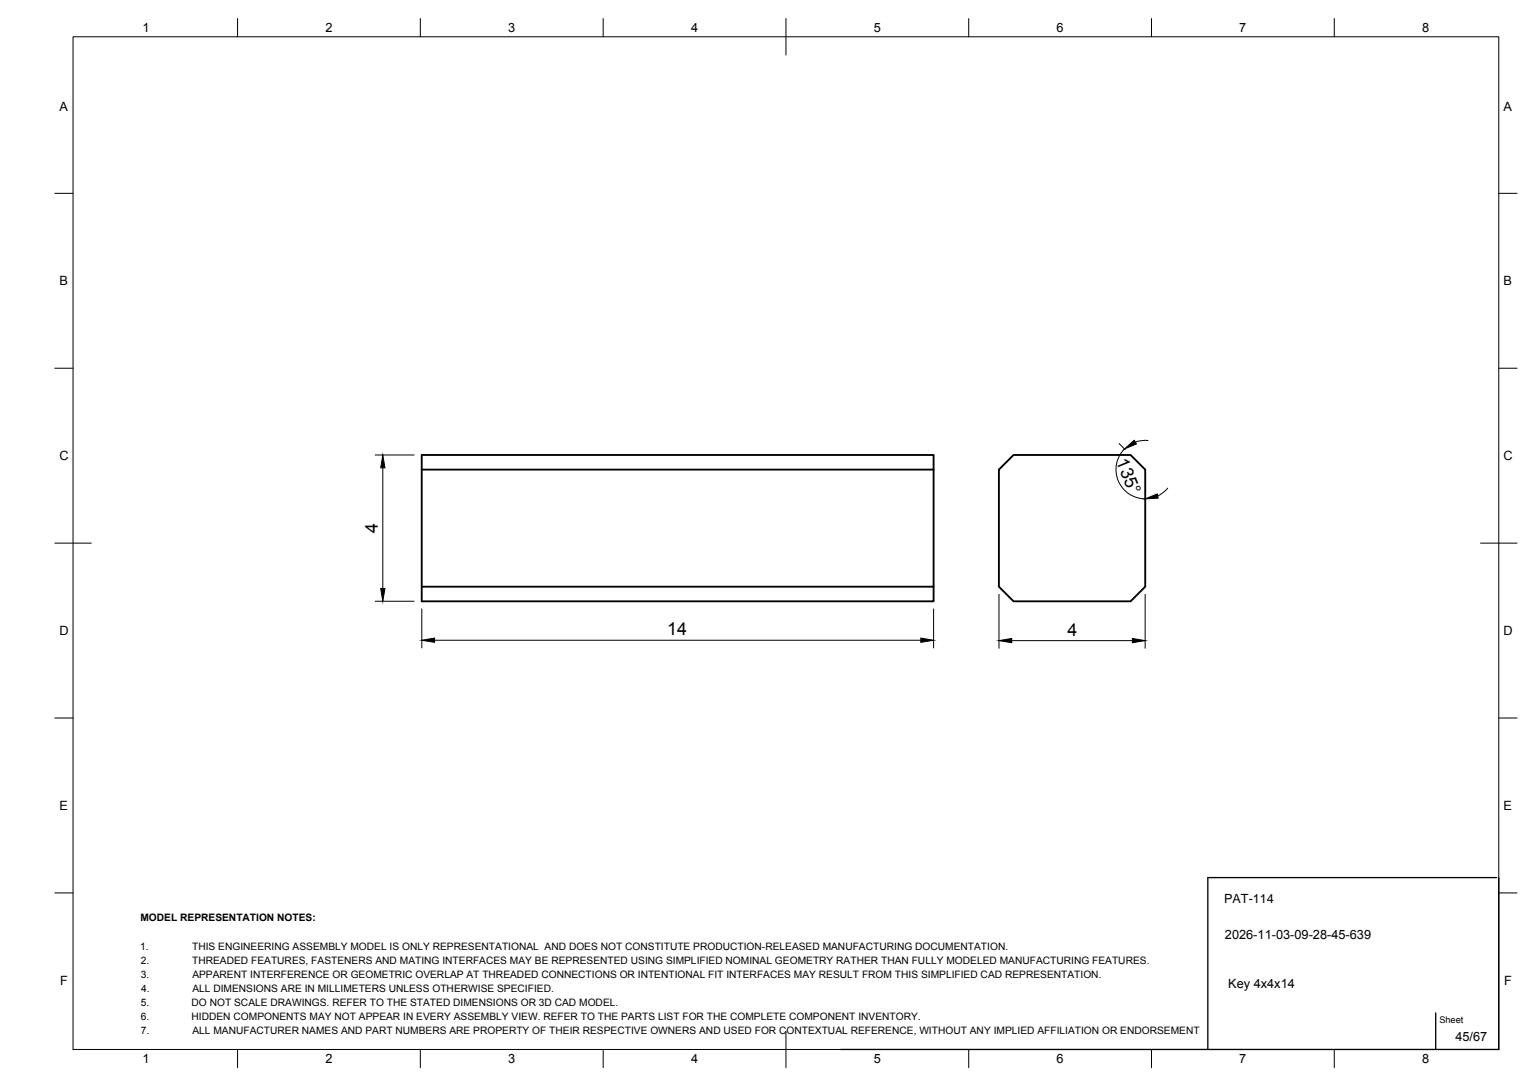
ISO-10303-21;
HEADER;
/* Generated by software containing ST-Developer
 * from STEP Tools, Inc. (www.steptools.com) 
 */

FILE_DESCRIPTION(
/* description */ ('Two-stage gear reducer in split housing'),
/* implementation_level */ '2;1');

FILE_NAME(
/* name */ 'Key 4x4x14.step',
/* time_stamp */ '2026-10-28T03:22:31-07:00',
/* author */ (''),
/* organization */ (''),
/* preprocessor_version */ 'ST-DEVELOPER v20.2',
/* originating_system */ 'Autodesk Translation Framework v15.17.0.0',
/* authorisation */ '');

FILE_SCHEMA (('AUTOMOTIVE_DESIGN { 1 0 10303 214 3 1 1 }'));
ENDSEC;

DATA;
#10=MECHANICAL_DESIGN_GEOMETRIC_PRESENTATION_REPRESENTATION('',(#1285),#73366);
#1158=SHAPE_REPRESENTATION_RELATIONSHIP('SRR','None',#73648,#1214);
#1214=ADVANCED_BREP_SHAPE_REPRESENTATION('',(#1354),#73344);
#1285=STYLED_ITEM('',(#73988),#1354);
#1354=MANIFOLD_SOLID_BREP('Body1',#16175);
#1848=PLANE('',#17938);
#1849=PLANE('',#17939);
#1850=PLANE('',#17940);
#1851=PLANE('',#17941);
#1852=PLANE('',#17942);
#1853=PLANE('',#17943);
#1854=PLANE('',#17944);
#1855=PLANE('',#17945);
#1856=PLANE('',#17946);
#1857=PLANE('',#17947);
#2542=FACE_OUTER_BOUND('',#3639,.T.);
#2543=FACE_OUTER_BOUND('',#3640,.T.);
#2544=FACE_OUTER_BOUND('',#3641,.T.);
#2545=FACE_OUTER_BOUND('',#3642,.T.);
#2546=FACE_OUTER_BOUND('',#3643,.T.);
#2547=FACE_OUTER_BOUND('',#3644,.T.);
#2548=FACE_OUTER_BOUND('',#3645,.T.);
#2549=FACE_OUTER_BOUND('',#3646,.T.);
#2550=FACE_OUTER_BOUND('',#3647,.T.);
#2551=FACE_OUTER_BOUND('',#3648,.T.);
#3639=EDGE_LOOP('',(#12941,#12942,#12943,#12944,#12945,#12946,#12947,#12948));
#3640=EDGE_LOOP('',(#12949,#12950,#12951,#12952));
#3641=EDGE_LOOP('',(#12953,#12954,#12955,#12956));
#3642=EDGE_LOOP('',(#12957,#12958,#12959,#12960));
#3643=EDGE_LOOP('',(#12961,#12962,#12963,#12964));
#3644=EDGE_LOOP('',(#12965,#12966,#12967,#12968,#12969,#12970,#12971,#12972));
#3645=EDGE_LOOP('',(#12973,#12974,#12975,#12976));
#3646=EDGE_LOOP('',(#12977,#12978,#12979,#12980));
#3647=EDGE_LOOP('',(#12981,#12982,#12983,#12984));
#3648=EDGE_LOOP('',(#12985,#12986,#12987,#12988));
#4639=LINE('',#37289,#5663);
#4640=LINE('',#37291,#5664);
#4641=LINE('',#37293,#5665);
#4642=LINE('',#37295,#5666);
#4643=LINE('',#37297,#5667);
#4644=LINE('',#37299,#5668);
#4645=LINE('',#37301,#5669);
#4646=LINE('',#37302,#5670);
#4647=LINE('',#37305,#5671);
#4648=LINE('',#37307,#5672);
#4649=LINE('',#37308,#5673);
#4650=LINE('',#37311,#5674);
#4651=LINE('',#37312,#5675);
#4652=LINE('',#37315,#5676);
#4653=LINE('',#37316,#5677);
#4654=LINE('',#37319,#5678);
#4655=LINE('',#37320,#5679);
#4656=LINE('',#37323,#5680);
#4657=LINE('',#37325,#5681);
#4658=LINE('',#37327,#5682);
#4659=LINE('',#37328,#5683);
#4660=LINE('',#37330,#5684);
#4661=LINE('',#37332,#5685);
#4662=LINE('',#37334,#5686);
#5663=VECTOR('',#21295,1.);
#5664=VECTOR('',#21296,1.);
#5665=VECTOR('',#21297,1.);
#5666=VECTOR('',#21298,1.);
#5667=VECTOR('',#21299,1.);
#5668=VECTOR('',#21300,1.);
#5669=VECTOR('',#21301,1.);
#5670=VECTOR('',#21302,1.);
#5671=VECTOR('',#21305,1.);
#5672=VECTOR('',#21306,1.);
#5673=VECTOR('',#21307,1.);
#5674=VECTOR('',#21310,1.);
#5675=VECTOR('',#21311,1.);
#5676=VECTOR('',#21314,1.);
#5677=VECTOR('',#21315,1.);
#5678=VECTOR('',#21318,1.);
#5679=VECTOR('',#21319,1.);
#5680=VECTOR('',#21322,1.);
#5681=VECTOR('',#21323,1.);
#5682=VECTOR('',#21324,1.);
#5683=VECTOR('',#21325,1.);
#5684=VECTOR('',#21328,1.);
#5685=VECTOR('',#21331,1.);
#5686=VECTOR('',#21334,1.);
#7651=VERTEX_POINT('',#37287);
#7652=VERTEX_POINT('',#37288);
#7653=VERTEX_POINT('',#37290);
#7654=VERTEX_POINT('',#37292);
#7655=VERTEX_POINT('',#37294);
#7656=VERTEX_POINT('',#37296);
#7657=VERTEX_POINT('',#37298);
#7658=VERTEX_POINT('',#37300);
#7659=VERTEX_POINT('',#37304);
#7660=VERTEX_POINT('',#37306);
#7661=VERTEX_POINT('',#37310);
#7662=VERTEX_POINT('',#37314);
#7663=VERTEX_POINT('',#37318);
#7664=VERTEX_POINT('',#37322);
#7665=VERTEX_POINT('',#37324);
#7666=VERTEX_POINT('',#37326);
#9524=EDGE_CURVE('',#7651,#7652,#4639,.T.);
#9525=EDGE_CURVE('',#7653,#7651,#4640,.T.);
#9526=EDGE_CURVE('',#7654,#7653,#4641,.T.);
#9527=EDGE_CURVE('',#7655,#7654,#4642,.T.);
#9528=EDGE_CURVE('',#7656,#7655,#4643,.T.);
#9529=EDGE_CURVE('',#7657,#7656,#4644,.T.);
#9530=EDGE_CURVE('',#7658,#7657,#4645,.T.);
#9531=EDGE_CURVE('',#7652,#7658,#4646,.T.);
#9532=EDGE_CURVE('',#7655,#7659,#4647,.T.);
#9533=EDGE_CURVE('',#7659,#7660,#4648,.T.);
#9534=EDGE_CURVE('',#7660,#7656,#4649,.T.);
#9535=EDGE_CURVE('',#7661,#7654,#4650,.T.);
#9536=EDGE_CURVE('',#7661,#7659,#4651,.T.);
#9537=EDGE_CURVE('',#7653,#7662,#4652,.T.);
#9538=EDGE_CURVE('',#7662,#7661,#4653,.T.);
#9539=EDGE_CURVE('',#7663,#7651,#4654,.T.);
#9540=EDGE_CURVE('',#7663,#7662,#4655,.T.);
#9541=EDGE_CURVE('',#7664,#7663,#4656,.T.);
#9542=EDGE_CURVE('',#7665,#7664,#4657,.T.);
#9543=EDGE_CURVE('',#7666,#7665,#4658,.T.);
#9544=EDGE_CURVE('',#7660,#7666,#4659,.T.);
#9545=EDGE_CURVE('',#7652,#7664,#4660,.T.);
#9546=EDGE_CURVE('',#7665,#7658,#4661,.T.);
#9547=EDGE_CURVE('',#7657,#7666,#4662,.T.);
#12941=ORIENTED_EDGE('',*,*,#9524,.F.);
#12942=ORIENTED_EDGE('',*,*,#9525,.F.);
#12943=ORIENTED_EDGE('',*,*,#9526,.F.);
#12944=ORIENTED_EDGE('',*,*,#9527,.F.);
#12945=ORIENTED_EDGE('',*,*,#9528,.F.);
#12946=ORIENTED_EDGE('',*,*,#9529,.F.);
#12947=ORIENTED_EDGE('',*,*,#9530,.F.);
#12948=ORIENTED_EDGE('',*,*,#9531,.F.);
#12949=ORIENTED_EDGE('',*,*,#9528,.T.);
#12950=ORIENTED_EDGE('',*,*,#9532,.T.);
#12951=ORIENTED_EDGE('',*,*,#9533,.T.);
#12952=ORIENTED_EDGE('',*,*,#9534,.T.);
#12953=ORIENTED_EDGE('',*,*,#9527,.T.);
#12954=ORIENTED_EDGE('',*,*,#9535,.F.);
#12955=ORIENTED_EDGE('',*,*,#9536,.T.);
#12956=ORIENTED_EDGE('',*,*,#9532,.F.);
#12957=ORIENTED_EDGE('',*,*,#9526,.T.);
#12958=ORIENTED_EDGE('',*,*,#9537,.T.);
#12959=ORIENTED_EDGE('',*,*,#9538,.T.);
#12960=ORIENTED_EDGE('',*,*,#9535,.T.);
#12961=ORIENTED_EDGE('',*,*,#9525,.T.);
#12962=ORIENTED_EDGE('',*,*,#9539,.F.);
#12963=ORIENTED_EDGE('',*,*,#9540,.T.);
#12964=ORIENTED_EDGE('',*,*,#9537,.F.);
#12965=ORIENTED_EDGE('',*,*,#9533,.F.);
#12966=ORIENTED_EDGE('',*,*,#9536,.F.);
#12967=ORIENTED_EDGE('',*,*,#9538,.F.);
#12968=ORIENTED_EDGE('',*,*,#9540,.F.);
#12969=ORIENTED_EDGE('',*,*,#9541,.F.);
#12970=ORIENTED_EDGE('',*,*,#9542,.F.);
#12971=ORIENTED_EDGE('',*,*,#9543,.F.);
#12972=ORIENTED_EDGE('',*,*,#9544,.F.);
#12973=ORIENTED_EDGE('',*,*,#9524,.T.);
#12974=ORIENTED_EDGE('',*,*,#9545,.T.);
#12975=ORIENTED_EDGE('',*,*,#9541,.T.);
#12976=ORIENTED_EDGE('',*,*,#9539,.T.);
#12977=ORIENTED_EDGE('',*,*,#9531,.T.);
#12978=ORIENTED_EDGE('',*,*,#9546,.F.);
#12979=ORIENTED_EDGE('',*,*,#9542,.T.);
#12980=ORIENTED_EDGE('',*,*,#9545,.F.);
#12981=ORIENTED_EDGE('',*,*,#9530,.T.);
#12982=ORIENTED_EDGE('',*,*,#9547,.T.);
#12983=ORIENTED_EDGE('',*,*,#9543,.T.);
#12984=ORIENTED_EDGE('',*,*,#9546,.T.);
#12985=ORIENTED_EDGE('',*,*,#9529,.T.);
#12986=ORIENTED_EDGE('',*,*,#9534,.F.);
#12987=ORIENTED_EDGE('',*,*,#9544,.T.);
#12988=ORIENTED_EDGE('',*,*,#9547,.F.);
#15749=ADVANCED_FACE('',(#2542),#1848,.T.);
#15750=ADVANCED_FACE('',(#2543),#1849,.T.);
#15751=ADVANCED_FACE('',(#2544),#1850,.T.);
#15752=ADVANCED_FACE('',(#2545),#1851,.T.);
#15753=ADVANCED_FACE('',(#2546),#1852,.T.);
#15754=ADVANCED_FACE('',(#2547),#1853,.F.);
#15755=ADVANCED_FACE('',(#2548),#1854,.T.);
#15756=ADVANCED_FACE('',(#2549),#1855,.T.);
#15757=ADVANCED_FACE('',(#2550),#1856,.T.);
#15758=ADVANCED_FACE('',(#2551),#1857,.F.);
#16175=CLOSED_SHELL('',(#15749,#15750,#15751,#15752,#15753,#15754,#15755,
#15756,#15757,#15758));
#17937=AXIS2_PLACEMENT_3D('',#37285,#21291,#21292);
#17938=AXIS2_PLACEMENT_3D('',#37286,#21293,#21294);
#17939=AXIS2_PLACEMENT_3D('',#37303,#21303,#21304);
#17940=AXIS2_PLACEMENT_3D('',#37309,#21308,#21309);
#17941=AXIS2_PLACEMENT_3D('',#37313,#21312,#21313);
#17942=AXIS2_PLACEMENT_3D('',#37317,#21316,#21317);
#17943=AXIS2_PLACEMENT_3D('',#37321,#21320,#21321);
#17944=AXIS2_PLACEMENT_3D('',#37329,#21326,#21327);
#17945=AXIS2_PLACEMENT_3D('',#37331,#21329,#21330);
#17946=AXIS2_PLACEMENT_3D('',#37333,#21332,#21333);
#17947=AXIS2_PLACEMENT_3D('',#37335,#21335,#21336);
#21291=DIRECTION('axis',(0.,0.,1.));
#21292=DIRECTION('refdir',(1.,0.,0.));
#21293=DIRECTION('center_axis',(1.,0.,0.));
#21294=DIRECTION('ref_axis',(0.,0.,-1.));
#21295=DIRECTION('',(0.,0.707106781186547,-0.707106781186548));
#21296=DIRECTION('',(0.,1.,0.));
#21297=DIRECTION('',(0.,0.707106781186547,0.707106781186548));
#21298=DIRECTION('',(0.,0.,1.));
#21299=DIRECTION('',(0.,-0.707106781186548,0.707106781186548));
#21300=DIRECTION('',(0.,-1.,0.));
#21301=DIRECTION('',(0.,-0.707106781186548,-0.707106781186548));
#21302=DIRECTION('',(0.,0.,-1.));
#21303=DIRECTION('center_axis',(0.,-0.707106781186548,-0.707106781186548));
#21304=DIRECTION('ref_axis',(-1.,0.,0.));
#21305=DIRECTION('',(-1.,0.,0.));
#21306=DIRECTION('',(0.,0.707106781186548,-0.707106781186548));
#21307=DIRECTION('',(1.,0.,0.));
#21308=DIRECTION('center_axis',(0.,-1.,0.));
#21309=DIRECTION('ref_axis',(1.,0.,0.));
#21310=DIRECTION('',(1.,0.,0.));
#21311=DIRECTION('',(0.,0.,-1.));
#21312=DIRECTION('center_axis',(0.,-0.707106781186548,0.707106781186547));
#21313=DIRECTION('ref_axis',(1.,0.,0.));
#21314=DIRECTION('',(-1.,0.,0.));
#21315=DIRECTION('',(0.,-0.707106781186547,-0.707106781186548));
#21316=DIRECTION('center_axis',(0.,0.,1.));
#21317=DIRECTION('ref_axis',(1.,0.,0.));
#21318=DIRECTION('',(1.,0.,0.));
#21319=DIRECTION('',(0.,-1.,0.));
#21320=DIRECTION('center_axis',(1.,0.,0.));
#21321=DIRECTION('ref_axis',(0.,0.,-1.));
#21322=DIRECTION('',(0.,-0.707106781186547,0.707106781186548));
#21323=DIRECTION('',(0.,0.,1.));
#21324=DIRECTION('',(0.,0.707106781186548,0.707106781186548));
#21325=DIRECTION('',(0.,1.,0.));
#21326=DIRECTION('center_axis',(0.,0.707106781186548,0.707106781186547));
#21327=DIRECTION('ref_axis',(1.,0.,0.));
#21328=DIRECTION('',(-1.,0.,0.));
#21329=DIRECTION('center_axis',(0.,1.,0.));
#21330=DIRECTION('ref_axis',(-1.,0.,0.));
#21331=DIRECTION('',(1.,0.,0.));
#21332=DIRECTION('center_axis',(0.,0.707106781186548,-0.707106781186548));
#21333=DIRECTION('ref_axis',(-1.,0.,0.));
#21334=DIRECTION('',(-1.,0.,0.));
#21335=DIRECTION('center_axis',(0.,0.,1.));
#21336=DIRECTION('ref_axis',(1.,0.,0.));
#37285=CARTESIAN_POINT('',(0.,0.,0.));
#37286=CARTESIAN_POINT('Origin',(0.7,0.,0.25));
#37287=CARTESIAN_POINT('',(0.7,0.16,0.4));
#37288=CARTESIAN_POINT('',(0.7,0.2,0.36));
#37289=CARTESIAN_POINT('',(0.7,0.1675,0.3925));
#37290=CARTESIAN_POINT('',(0.7,-0.16,0.4));
#37291=CARTESIAN_POINT('',(0.7,0.,0.4));
#37292=CARTESIAN_POINT('',(0.7,-0.2,0.36));
#37293=CARTESIAN_POINT('',(0.7,-0.1675,0.3925));
#37294=CARTESIAN_POINT('',(0.7,-0.2,0.04));
#37295=CARTESIAN_POINT('',(0.7,-0.2,0.125));
#37296=CARTESIAN_POINT('',(0.7,-0.16,0.));
#37297=CARTESIAN_POINT('',(0.7,-0.1925,0.0325));
#37298=CARTESIAN_POINT('',(0.7,0.16,0.));
#37299=CARTESIAN_POINT('',(0.7,0.,0.));
#37300=CARTESIAN_POINT('',(0.7,0.2,0.04));
#37301=CARTESIAN_POINT('',(0.7,0.1925,0.0325));
#37302=CARTESIAN_POINT('',(0.7,0.2,0.125));
#37303=CARTESIAN_POINT('Origin',(-0.4,-0.18,0.02));
#37304=CARTESIAN_POINT('',(-0.7,-0.2,0.04));
#37305=CARTESIAN_POINT('',(-0.4,-0.2,0.04));
#37306=CARTESIAN_POINT('',(-0.7,-0.16,0.));
#37307=CARTESIAN_POINT('',(-0.7,-0.1925,0.0325));
#37308=CARTESIAN_POINT('',(-0.4,-0.16,0.));
#37309=CARTESIAN_POINT('Origin',(-0.8,-0.2,0.));
#37310=CARTESIAN_POINT('',(-0.7,-0.2,0.36));
#37311=CARTESIAN_POINT('',(-0.4,-0.2,0.36));
#37312=CARTESIAN_POINT('',(-0.7,-0.2,0.125));
#37313=CARTESIAN_POINT('Origin',(-0.4,-0.18,0.38));
#37314=CARTESIAN_POINT('',(-0.7,-0.16,0.4));
#37315=CARTESIAN_POINT('',(-0.4,-0.16,0.4));
#37316=CARTESIAN_POINT('',(-0.7,-0.1675,0.3925));
#37317=CARTESIAN_POINT('Origin',(0.,0.,0.4));
#37318=CARTESIAN_POINT('',(-0.7,0.16,0.4));
#37319=CARTESIAN_POINT('',(0.4,0.16,0.4));
#37320=CARTESIAN_POINT('',(-0.7,0.,0.4));
#37321=CARTESIAN_POINT('Origin',(-0.7,0.,0.25));
#37322=CARTESIAN_POINT('',(-0.7,0.2,0.36));
#37323=CARTESIAN_POINT('',(-0.7,0.1675,0.3925));
#37324=CARTESIAN_POINT('',(-0.7,0.2,0.04));
#37325=CARTESIAN_POINT('',(-0.7,0.2,0.125));
#37326=CARTESIAN_POINT('',(-0.7,0.16,0.));
#37327=CARTESIAN_POINT('',(-0.7,0.1925,0.0325));
#37328=CARTESIAN_POINT('',(-0.7,0.,0.));
#37329=CARTESIAN_POINT('Origin',(0.4,0.18,0.38));
#37330=CARTESIAN_POINT('',(0.4,0.2,0.36));
#37331=CARTESIAN_POINT('Origin',(0.8,0.2,0.));
#37332=CARTESIAN_POINT('',(0.4,0.2,0.04));
#37333=CARTESIAN_POINT('Origin',(0.4,0.18,0.02));
#37334=CARTESIAN_POINT('',(0.4,0.16,0.));
#37335=CARTESIAN_POINT('Origin',(0.,0.,0.));
#73280=UNCERTAINTY_MEASURE_WITH_UNIT(LENGTH_MEASURE(0.001),#73367,
'DISTANCE_ACCURACY_VALUE',
'Maximum model space distance between geometric entities at asserted c
onnectivities');
#73302=UNCERTAINTY_MEASURE_WITH_UNIT(LENGTH_MEASURE(0.001),#73367,
'DISTANCE_ACCURACY_VALUE',
'Maximum model space distance between geometric entities at asserted c
onnectivities');
#73344=(
GEOMETRIC_REPRESENTATION_CONTEXT(3)
GLOBAL_UNCERTAINTY_ASSIGNED_CONTEXT((#73280))
GLOBAL_UNIT_ASSIGNED_CONTEXT((#73367,#73369,#73370))
REPRESENTATION_CONTEXT('','3D')
);
#73366=(
GEOMETRIC_REPRESENTATION_CONTEXT(3)
GLOBAL_UNCERTAINTY_ASSIGNED_CONTEXT((#73302))
GLOBAL_UNIT_ASSIGNED_CONTEXT((#73367,#73369,#73370))
REPRESENTATION_CONTEXT('','3D')
);
#73367=(
LENGTH_UNIT()
NAMED_UNIT(*)
SI_UNIT(.CENTI.,.METRE.)
);
#73369=(
NAMED_UNIT(*)
PLANE_ANGLE_UNIT()
SI_UNIT($,.RADIAN.)
);
#73370=(
NAMED_UNIT(*)
SI_UNIT($,.STERADIAN.)
SOLID_ANGLE_UNIT()
);
#73412=SHAPE_DEFINITION_REPRESENTATION(#73545,#73648);
#73545=PRODUCT_DEFINITION_SHAPE('',$,#73712);
#73648=SHAPE_REPRESENTATION('',(#17937),#73344);
#73670=PRODUCT_DEFINITION_CONTEXT('part definition',#73861,'design');
#73712=PRODUCT_DEFINITION('Key 4x4x14','Key 4x4x14',#73775,#73670);
#73775=PRODUCT_DEFINITION_FORMATION('',$,#73904);
#73861=APPLICATION_CONTEXT(
'Core Data for Automotive Mechanical Design Process');
#73862=PRODUCT_CONTEXT('part definition',#73861,'mechanical');
#73904=PRODUCT('Key 4x4x14','Key 4x4x14','Key 4x4x14',(#73862));
#73982=COLOUR_RGB('Grey',0.48,0.52,0.57);
#73983=FILL_AREA_STYLE_COLOUR('',#73982);
#73984=FILL_AREA_STYLE('',(#73983));
#73985=SURFACE_STYLE_FILL_AREA(#73984);
#73986=SURFACE_SIDE_STYLE('',(#73985));
#73987=SURFACE_STYLE_USAGE(.BOTH.,#73986);
#73988=PRESENTATION_STYLE_ASSIGNMENT((#73987));
ENDSEC;
END-ISO-10303-21;
